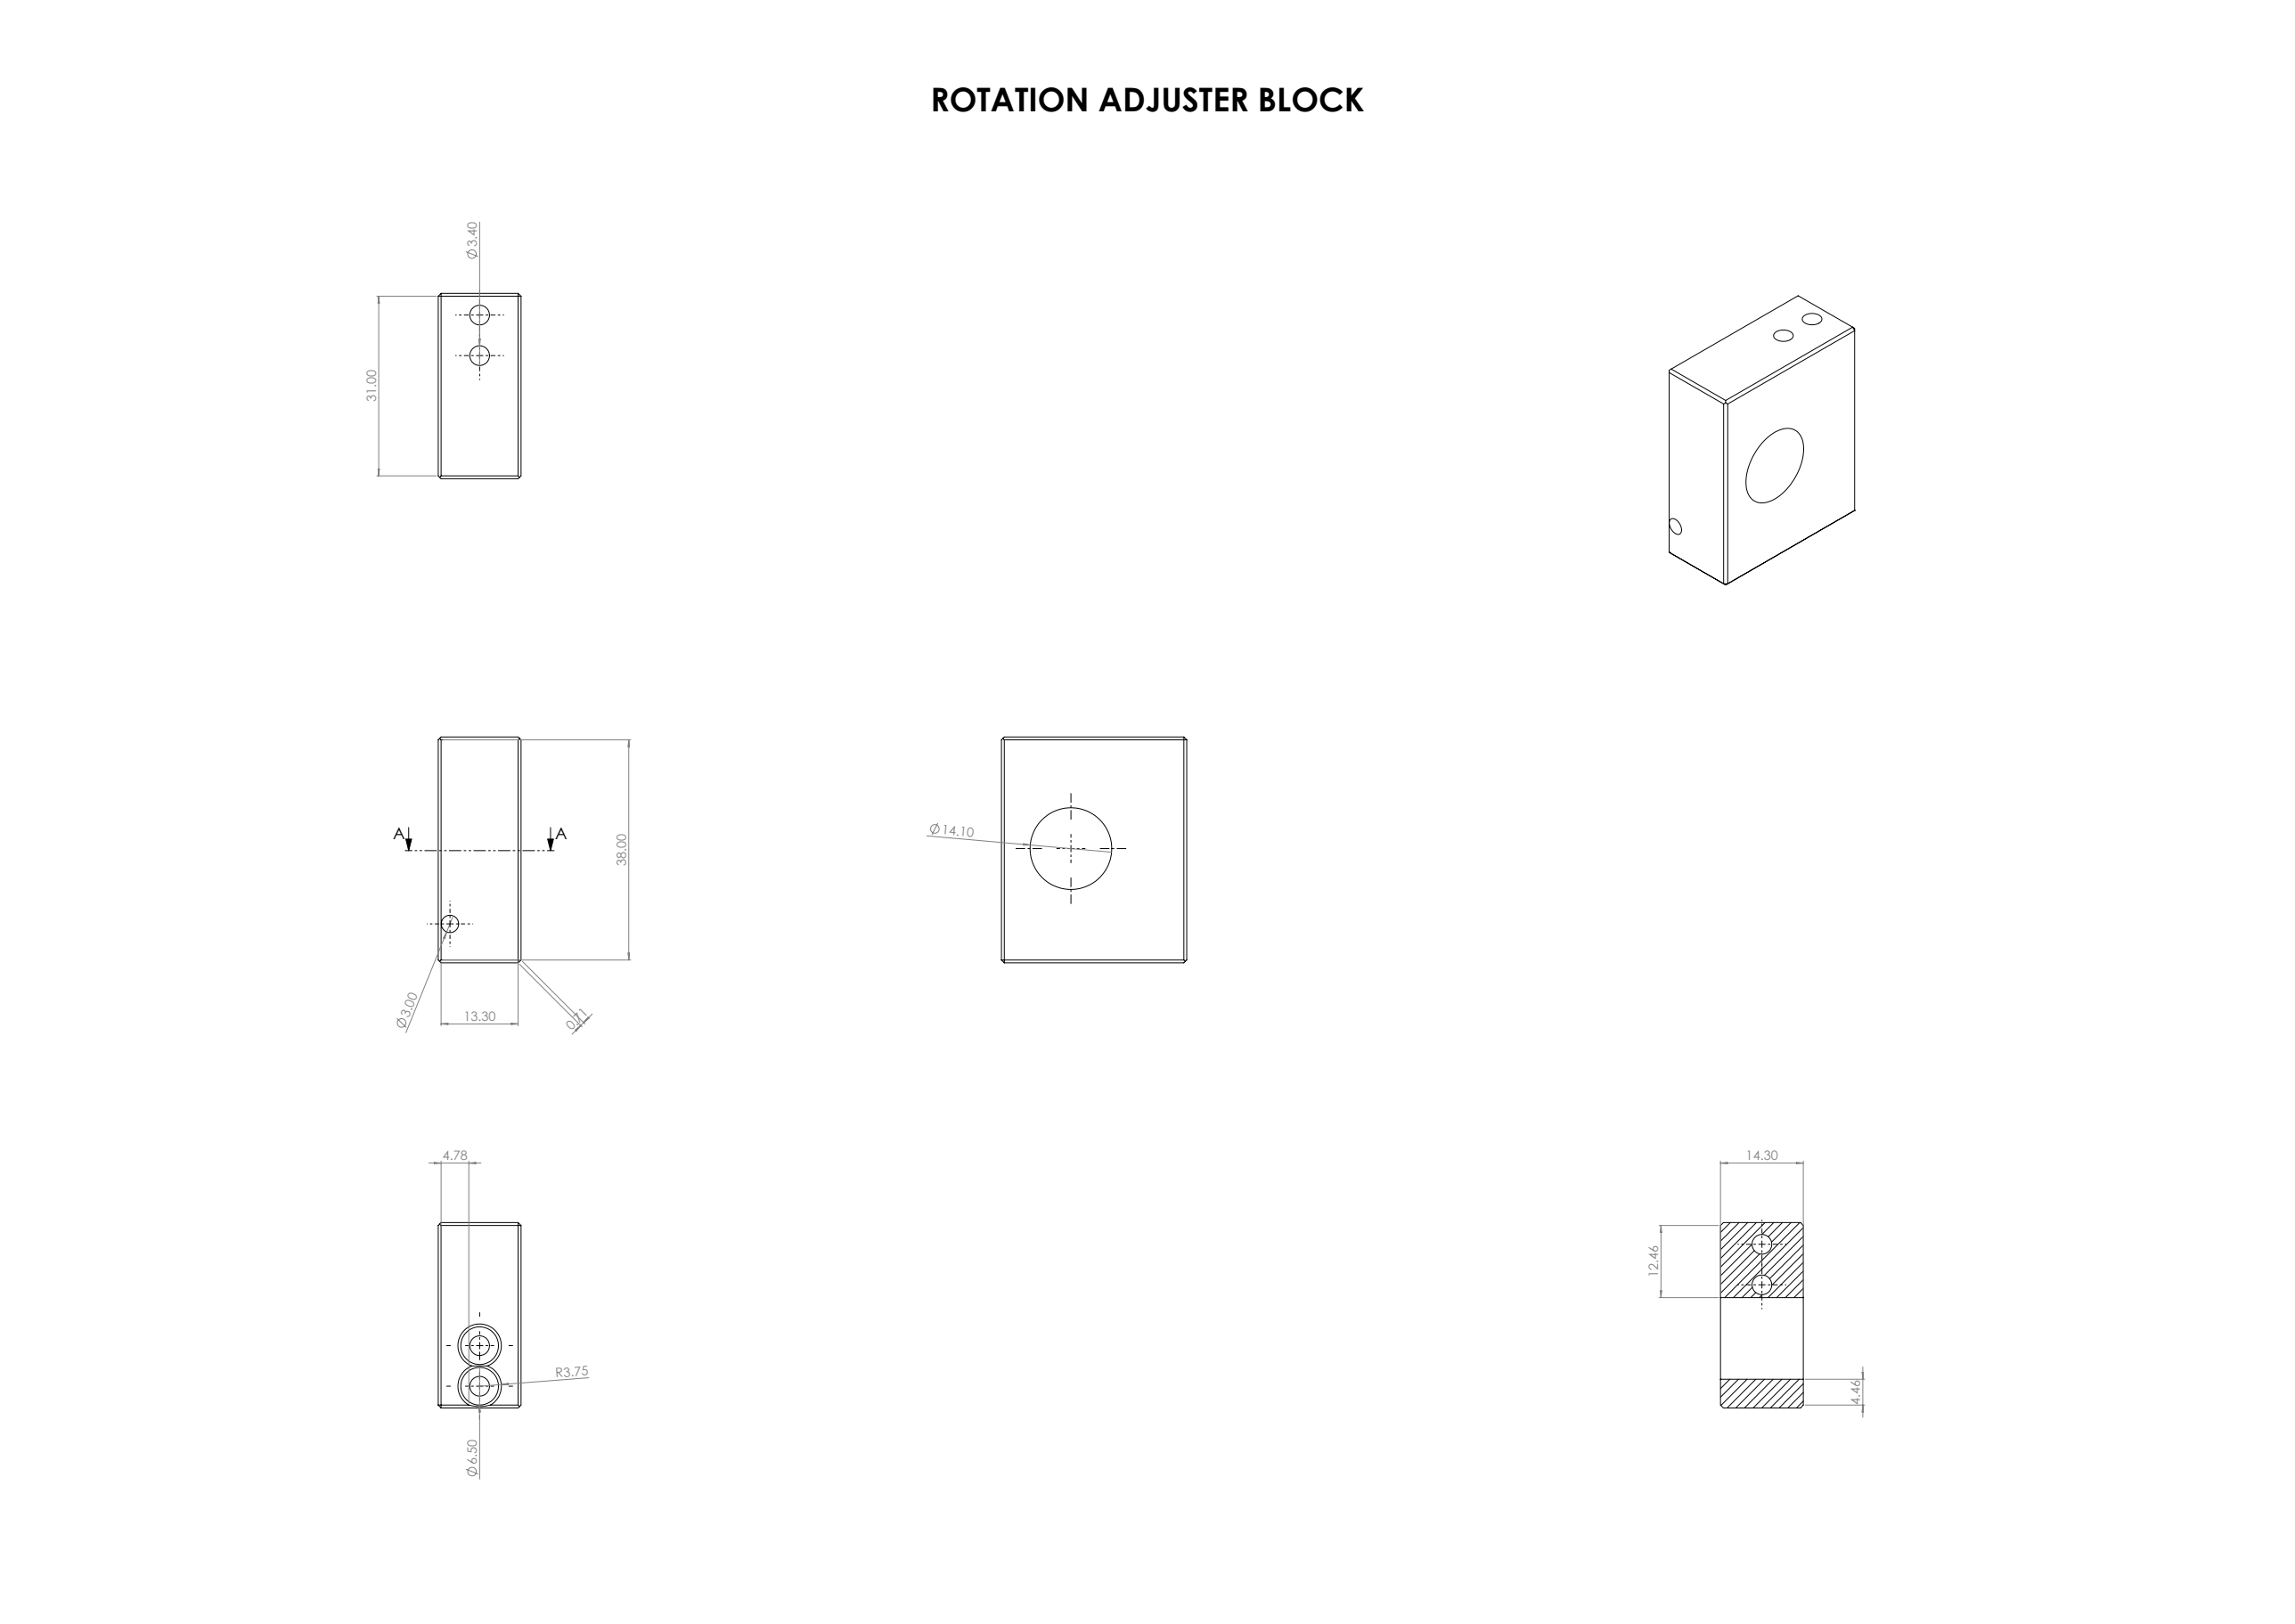
ISO-10303-21;
HEADER;
/* Generated by software containing ST-Developer
 * from STEP Tools, Inc. (www.steptools.com) 
 */

FILE_DESCRIPTION(
/* description */ (''),
/* implementation_level */ '2;1');

FILE_NAME(
/* name */ '04_Rotation_Adjuster_Block.step',
/* time_stamp */ '2026-10-21T01:56:51-07:00',
/* author */ (''),
/* organization */ (''),
/* preprocessor_version */ 'ST-DEVELOPER v20.2',
/* originating_system */ 'Autodesk Translation Framework v15.15.0.0',
/* authorisation */ '');

FILE_SCHEMA (('AUTOMOTIVE_DESIGN { 1 0 10303 214 3 1 1 }'));
ENDSEC;

DATA;
#10=MECHANICAL_DESIGN_GEOMETRIC_PRESENTATION_REPRESENTATION('',(#273),#82384);
#169=(
BOUNDED_CURVE()
B_SPLINE_CURVE(2,(#44591,#44592,#44593),.UNSPECIFIED.,.F.,.F.)
B_SPLINE_CURVE_WITH_KNOTS((3,3),(0.,0.380788655293197),.UNSPECIFIED.)
CURVE()
GEOMETRIC_REPRESENTATION_ITEM()
RATIONAL_B_SPLINE_CURVE((1.,1.,1.))
REPRESENTATION_ITEM('')
);
#235=SHAPE_REPRESENTATION_RELATIONSHIP('SRR','None',#82469,#254);
#254=ADVANCED_BREP_SHAPE_REPRESENTATION('',(#292),#82368);
#273=STYLED_ITEM('',(#82610),#292);
#292=MANIFOLD_SOLID_BREP('Body1',#30664);
#538=CYLINDRICAL_SURFACE('',#31720,3.25);
#539=CYLINDRICAL_SURFACE('',#31723,3.25);
#540=CYLINDRICAL_SURFACE('',#31755,1.7);
#541=CYLINDRICAL_SURFACE('',#31756,1.7);
#542=CYLINDRICAL_SURFACE('',#31757,1.5);
#543=CYLINDRICAL_SURFACE('',#31758,1.5);
#544=CYLINDRICAL_SURFACE('',#31761,4.5);
#545=CYLINDRICAL_SURFACE('',#31764,7.05);
#1402=CIRCLE('',#31712,3.75);
#1403=CIRCLE('',#31713,3.25);
#1404=CIRCLE('',#31714,3.75);
#1405=CIRCLE('',#31716,3.75);
#1406=CIRCLE('',#31717,3.25);
#1407=CIRCLE('',#31718,3.75);
#1408=CIRCLE('',#31719,3.75);
#1409=CIRCLE('',#31721,3.25);
#1410=CIRCLE('',#31724,3.25);
#1411=CIRCLE('',#31735,1.7);
#1412=CIRCLE('',#31736,1.7);
#1413=CIRCLE('',#31738,7.05);
#1414=CIRCLE('',#31739,4.5);
#1415=CIRCLE('',#31748,7.05);
#1416=CIRCLE('',#31750,1.5);
#1417=CIRCLE('',#31752,1.7);
#1418=CIRCLE('',#31754,1.7);
#1419=CIRCLE('',#31759,1.5);
#1420=CIRCLE('',#31762,4.5);
#2029=CONICAL_SURFACE('',#31711,3.5,0.785398163397442);
#2030=CONICAL_SURFACE('',#31715,3.5,0.785398163397442);
#2310=B_SPLINE_CURVE_WITH_KNOTS('',3,(#44570,#44571,#44572,#44573,#44574,
#44575),.UNSPECIFIED.,.F.,.F.,(4,2,4),(1.60159343096041,1.75059102484718,
1.89958861873394),.UNSPECIFIED.);
#2311=B_SPLINE_CURVE_WITH_KNOTS('',3,(#44727,#44728,#44729,#44730,#44731,
#44732,#44733,#44734,#44735,#44736),.UNSPECIFIED.,.F.,.F.,(4,2,2,2,4),(0.,
0.056990727183553,0.113981454367106,0.170945749207414,0.227910044047722),
 .UNSPECIFIED.);
#2312=B_SPLINE_CURVE_WITH_KNOTS('',3,(#44738,#44739,#44740,#44741,#44742,
#44743,#44744,#44745,#44746,#44747),.UNSPECIFIED.,.F.,.F.,(4,2,2,2,4),(0.683730132143166,
0.740694426983474,0.797658721823782,0.854649449007335,0.911640176190888),
 .UNSPECIFIED.);
#2313=B_SPLINE_CURVE_WITH_KNOTS('',3,(#44748,#44749,#44750,#44751,#44752,
#44753,#44754,#44755,#44756,#44757,#44758,#44759,#44760,#44761,#44762,#44763,
#44764,#44765),.UNSPECIFIED.,.F.,.F.,(4,2,2,2,2,2,2,2,4),(0.227910044047722,
0.28487433888803,0.341838633728338,0.398829360911891,0.455820088095444,
0.512810815278997,0.56980154246255,0.626765837302858,0.683730132143166),
 .UNSPECIFIED.);
#2314=B_SPLINE_CURVE_WITH_KNOTS('',3,(#44769,#44770,#44771,#44772,#44773,
#44774,#44775,#44776,#44777,#44778,#44779,#44780,#44781,#44782,#44783,#44784,
#44785,#44786,#44787,#44788,#44789,#44790,#44791,#44792,#44793,#44794),
 .UNSPECIFIED.,.F.,.F.,(4,2,2,2,2,2,2,2,2,2,2,2,4),(0.,0.056990727183553,
0.113981454367106,0.170945749207414,0.227910044047722,0.28487433888803,
0.341838633728338,0.398829360911891,0.455820088095444,0.512810815278997,
0.56980154246255,0.626765837302858,0.683730132143166),.UNSPECIFIED.);
#2315=B_SPLINE_CURVE_WITH_KNOTS('',3,(#44795,#44796,#44797,#44798,#44799,
#44800,#44801,#44802,#44803,#44804),.UNSPECIFIED.,.F.,.F.,(4,2,2,2,4),(0.683730132143166,
0.740694426983474,0.797658721823782,0.854649449007335,0.911640176190888),
 .UNSPECIFIED.);
#3434=FACE_BOUND('',#6058,.T.);
#3435=FACE_BOUND('',#6059,.T.);
#3436=FACE_BOUND('',#6061,.T.);
#3437=FACE_BOUND('',#6062,.T.);
#3438=FACE_BOUND('',#6071,.T.);
#3439=FACE_BOUND('',#6073,.T.);
#3440=FACE_BOUND('',#6075,.T.);
#3441=FACE_BOUND('',#6077,.T.);
#3442=FACE_BOUND('',#6084,.T.);
#4137=FACE_OUTER_BOUND('',#6043,.T.);
#4138=FACE_OUTER_BOUND('',#6044,.T.);
#4139=FACE_OUTER_BOUND('',#6045,.T.);
#4140=FACE_OUTER_BOUND('',#6046,.T.);
#4141=FACE_OUTER_BOUND('',#6047,.T.);
#4142=FACE_OUTER_BOUND('',#6048,.T.);
#4143=FACE_OUTER_BOUND('',#6049,.T.);
#4144=FACE_OUTER_BOUND('',#6050,.T.);
#4145=FACE_OUTER_BOUND('',#6051,.T.);
#4146=FACE_OUTER_BOUND('',#6052,.T.);
#4147=FACE_OUTER_BOUND('',#6053,.T.);
#4148=FACE_OUTER_BOUND('',#6054,.T.);
#4149=FACE_OUTER_BOUND('',#6055,.T.);
#4150=FACE_OUTER_BOUND('',#6056,.T.);
#4151=FACE_OUTER_BOUND('',#6057,.T.);
#4152=FACE_OUTER_BOUND('',#6060,.T.);
#4153=FACE_OUTER_BOUND('',#6063,.T.);
#4154=FACE_OUTER_BOUND('',#6064,.T.);
#4155=FACE_OUTER_BOUND('',#6065,.T.);
#4156=FACE_OUTER_BOUND('',#6066,.T.);
#4157=FACE_OUTER_BOUND('',#6067,.T.);
#4158=FACE_OUTER_BOUND('',#6068,.T.);
#4159=FACE_OUTER_BOUND('',#6069,.T.);
#4160=FACE_OUTER_BOUND('',#6070,.T.);
#4161=FACE_OUTER_BOUND('',#6072,.T.);
#4162=FACE_OUTER_BOUND('',#6074,.T.);
#4163=FACE_OUTER_BOUND('',#6076,.T.);
#4164=FACE_OUTER_BOUND('',#6078,.T.);
#4165=FACE_OUTER_BOUND('',#6079,.T.);
#4166=FACE_OUTER_BOUND('',#6080,.T.);
#4167=FACE_OUTER_BOUND('',#6081,.T.);
#4168=FACE_OUTER_BOUND('',#6082,.T.);
#4169=FACE_OUTER_BOUND('',#6083,.T.);
#4170=FACE_OUTER_BOUND('',#6085,.T.);
#4171=FACE_OUTER_BOUND('',#6086,.T.);
#4172=FACE_OUTER_BOUND('',#6087,.T.);
#6043=EDGE_LOOP('',(#21929,#21930,#21931,#21932,#21933,#21934));
#6044=EDGE_LOOP('',(#21935,#21936,#21937,#21938,#21939,#21940,#21941,#21942));
#6045=EDGE_LOOP('',(#21943,#21944,#21945,#21946));
#6046=EDGE_LOOP('',(#21947,#21948,#21949,#21950,#21951,#21952,#21953));
#6047=EDGE_LOOP('',(#21954,#21955,#21956,#21957));
#6048=EDGE_LOOP('',(#21958,#21959,#21960));
#6049=EDGE_LOOP('',(#21961,#21962,#21963));
#6050=EDGE_LOOP('',(#21964,#21965,#21966,#21967));
#6051=EDGE_LOOP('',(#21968,#21969,#21970,#21971,#21972));
#6052=EDGE_LOOP('',(#21973,#21974,#21975));
#6053=EDGE_LOOP('',(#21976,#21977,#21978,#21979,#21980));
#6054=EDGE_LOOP('',(#21981,#21982,#21983,#21984));
#6055=EDGE_LOOP('',(#21985,#21986,#21987,#21988,#21989));
#6056=EDGE_LOOP('',(#21990,#21991,#21992,#21993,#21994));
#6057=EDGE_LOOP('',(#21995,#21996,#21997,#21998));
#6058=EDGE_LOOP('',(#21999));
#6059=EDGE_LOOP('',(#22000));
#6060=EDGE_LOOP('',(#22001,#22002,#22003,#22004));
#6061=EDGE_LOOP('',(#22005));
#6062=EDGE_LOOP('',(#22006));
#6063=EDGE_LOOP('',(#22007,#22008,#22009,#22010,#22011,#22012));
#6064=EDGE_LOOP('',(#22013,#22014,#22015,#22016,#22017));
#6065=EDGE_LOOP('',(#22018,#22019,#22020,#22021));
#6066=EDGE_LOOP('',(#22022,#22023,#22024));
#6067=EDGE_LOOP('',(#22025,#22026,#22027,#22028,#22029));
#6068=EDGE_LOOP('',(#22030,#22031,#22032,#22033,#22034,#22035));
#6069=EDGE_LOOP('',(#22036,#22037,#22038,#22039,#22040));
#6070=EDGE_LOOP('',(#22041,#22042,#22043,#22044));
#6071=EDGE_LOOP('',(#22045));
#6072=EDGE_LOOP('',(#22046,#22047,#22048,#22049));
#6073=EDGE_LOOP('',(#22050));
#6074=EDGE_LOOP('',(#22051));
#6075=EDGE_LOOP('',(#22052));
#6076=EDGE_LOOP('',(#22053));
#6077=EDGE_LOOP('',(#22054));
#6078=EDGE_LOOP('',(#22055,#22056,#22057,#22058));
#6079=EDGE_LOOP('',(#22059,#22060,#22061,#22062));
#6080=EDGE_LOOP('',(#22063,#22064,#22065,#22066,#22067,#22068));
#6081=EDGE_LOOP('',(#22069,#22070,#22071,#22072,#22073));
#6082=EDGE_LOOP('',(#22074));
#6083=EDGE_LOOP('',(#22075,#22076,#22077,#22078,#22079,#22080,#22081,#22082,
#22083));
#6084=EDGE_LOOP('',(#22084,#22085));
#6085=EDGE_LOOP('',(#22086));
#6086=EDGE_LOOP('',(#22087,#22088,#22089,#22090));
#6087=EDGE_LOOP('',(#22091,#22092,#22093,#22094,#22095,#22096,#22097,#22098,
#22099,#22100));
#8112=LINE('',#44579,#10418);
#8113=LINE('',#44586,#10419);
#8114=LINE('',#44597,#10420);
#8115=LINE('',#44601,#10421);
#8116=LINE('',#44603,#10422);
#8117=LINE('',#44605,#10423);
#8118=LINE('',#44607,#10424);
#8119=LINE('',#44609,#10425);
#8120=LINE('',#44610,#10426);
#8121=LINE('',#44613,#10427);
#8122=LINE('',#44617,#10428);
#8123=LINE('',#44618,#10429);
#8124=LINE('',#44622,#10430);
#8125=LINE('',#44624,#10431);
#8126=LINE('',#44625,#10432);
#8127=LINE('',#44627,#10433);
#8128=LINE('',#44628,#10434);
#8129=LINE('',#44632,#10435);
#8130=LINE('',#44633,#10436);
#8131=LINE('',#44635,#10437);
#8132=LINE('',#44636,#10438);
#8133=LINE('',#44640,#10439);
#8134=LINE('',#44642,#10440);
#8135=LINE('',#44643,#10441);
#8136=LINE('',#44645,#10442);
#8137=LINE('',#44647,#10443);
#8138=LINE('',#44648,#10444);
#8139=LINE('',#44650,#10445);
#8140=LINE('',#44651,#10446);
#8141=LINE('',#44655,#10447);
#8142=LINE('',#44656,#10448);
#8143=LINE('',#44658,#10449);
#8144=LINE('',#44659,#10450);
#8145=LINE('',#44663,#10451);
#8146=LINE('',#44664,#10452);
#8147=LINE('',#44666,#10453);
#8148=LINE('',#44667,#10454);
#8149=LINE('',#44669,#10455);
#8150=LINE('',#44675,#10456);
#8151=LINE('',#44682,#10457);
#8152=LINE('',#44684,#10458);
#8153=LINE('',#44685,#10459);
#8154=LINE('',#44688,#10460);
#8155=LINE('',#44690,#10461);
#8156=LINE('',#44691,#10462);
#8157=LINE('',#44695,#10463);
#8158=LINE('',#44696,#10464);
#8159=LINE('',#44698,#10465);
#8160=LINE('',#44699,#10466);
#8161=LINE('',#44702,#10467);
#8162=LINE('',#44703,#10468);
#8163=LINE('',#44705,#10469);
#8164=LINE('',#44706,#10470);
#8165=LINE('',#44720,#10471);
#8166=LINE('',#44722,#10472);
#8167=LINE('',#44725,#10473);
#8168=LINE('',#44806,#10474);
#8169=LINE('',#44810,#10475);
#8170=LINE('',#44812,#10476);
#8171=LINE('',#44816,#10477);
#10418=VECTOR('',#35789,3.5);
#10419=VECTOR('',#35798,3.5);
#10420=VECTOR('',#35807,3.25);
#10421=VECTOR('',#35812,10.);
#10422=VECTOR('',#35813,10.);
#10423=VECTOR('',#35814,10.);
#10424=VECTOR('',#35815,10.);
#10425=VECTOR('',#35816,10.);
#10426=VECTOR('',#35817,10.);
#10427=VECTOR('',#35820,3.25);
#10428=VECTOR('',#35825,10.);
#10429=VECTOR('',#35826,10.);
#10430=VECTOR('',#35829,10.);
#10431=VECTOR('',#35830,10.);
#10432=VECTOR('',#35831,10.);
#10433=VECTOR('',#35834,10.);
#10434=VECTOR('',#35835,10.);
#10435=VECTOR('',#35838,10.);
#10436=VECTOR('',#35839,10.);
#10437=VECTOR('',#35840,10.);
#10438=VECTOR('',#35841,10.);
#10439=VECTOR('',#35844,10.);
#10440=VECTOR('',#35845,10.);
#10441=VECTOR('',#35846,10.);
#10442=VECTOR('',#35849,10.);
#10443=VECTOR('',#35850,10.);
#10444=VECTOR('',#35851,10.);
#10445=VECTOR('',#35854,10.);
#10446=VECTOR('',#35855,10.);
#10447=VECTOR('',#35858,10.);
#10448=VECTOR('',#35859,10.);
#10449=VECTOR('',#35860,10.);
#10450=VECTOR('',#35861,10.);
#10451=VECTOR('',#35864,10.);
#10452=VECTOR('',#35865,10.);
#10453=VECTOR('',#35866,10.);
#10454=VECTOR('',#35867,10.);
#10455=VECTOR('',#35870,10.);
#10456=VECTOR('',#35877,10.);
#10457=VECTOR('',#35884,10.);
#10458=VECTOR('',#35885,10.);
#10459=VECTOR('',#35886,10.);
#10460=VECTOR('',#35889,10.);
#10461=VECTOR('',#35890,10.);
#10462=VECTOR('',#35891,10.);
#10463=VECTOR('',#35896,10.);
#10464=VECTOR('',#35897,10.);
#10465=VECTOR('',#35900,10.);
#10466=VECTOR('',#35901,10.);
#10467=VECTOR('',#35904,10.);
#10468=VECTOR('',#35905,10.);
#10469=VECTOR('',#35908,10.);
#10470=VECTOR('',#35909,10.);
#10471=VECTOR('',#35928,1.7);
#10472=VECTOR('',#35931,1.7);
#10473=VECTOR('',#35934,1.5);
#10474=VECTOR('',#35937,1.5);
#10475=VECTOR('',#35944,4.5);
#10476=VECTOR('',#35945,4.5);
#10477=VECTOR('',#35952,7.05);
#12816=VERTEX_POINT('',#44568);
#12817=VERTEX_POINT('',#44569);
#12818=VERTEX_POINT('',#44576);
#12819=VERTEX_POINT('',#44578);
#12820=VERTEX_POINT('',#44583);
#12821=VERTEX_POINT('',#44585);
#12822=VERTEX_POINT('',#44588);
#12823=VERTEX_POINT('',#44590);
#12824=VERTEX_POINT('',#44596);
#12825=VERTEX_POINT('',#44600);
#12826=VERTEX_POINT('',#44602);
#12827=VERTEX_POINT('',#44604);
#12828=VERTEX_POINT('',#44606);
#12829=VERTEX_POINT('',#44608);
#12830=VERTEX_POINT('',#44612);
#12831=VERTEX_POINT('',#44616);
#12832=VERTEX_POINT('',#44620);
#12833=VERTEX_POINT('',#44621);
#12834=VERTEX_POINT('',#44623);
#12835=VERTEX_POINT('',#44630);
#12836=VERTEX_POINT('',#44631);
#12837=VERTEX_POINT('',#44634);
#12838=VERTEX_POINT('',#44638);
#12839=VERTEX_POINT('',#44639);
#12840=VERTEX_POINT('',#44641);
#12841=VERTEX_POINT('',#44646);
#12842=VERTEX_POINT('',#44653);
#12843=VERTEX_POINT('',#44654);
#12844=VERTEX_POINT('',#44657);
#12845=VERTEX_POINT('',#44661);
#12846=VERTEX_POINT('',#44662);
#12847=VERTEX_POINT('',#44665);
#12848=VERTEX_POINT('',#44670);
#12849=VERTEX_POINT('',#44672);
#12850=VERTEX_POINT('',#44676);
#12851=VERTEX_POINT('',#44678);
#12852=VERTEX_POINT('',#44681);
#12853=VERTEX_POINT('',#44683);
#12854=VERTEX_POINT('',#44687);
#12855=VERTEX_POINT('',#44689);
#12856=VERTEX_POINT('',#44694);
#12857=VERTEX_POINT('',#44701);
#12858=VERTEX_POINT('',#44708);
#12859=VERTEX_POINT('',#44711);
#12860=VERTEX_POINT('',#44714);
#12861=VERTEX_POINT('',#44717);
#12862=VERTEX_POINT('',#44724);
#12863=VERTEX_POINT('',#44726);
#12864=VERTEX_POINT('',#44737);
#12865=VERTEX_POINT('',#44767);
#12866=VERTEX_POINT('',#44768);
#12867=VERTEX_POINT('',#44805);
#12868=VERTEX_POINT('',#44811);
#16186=EDGE_CURVE('',#12816,#12817,#2310,.T.);
#16187=EDGE_CURVE('',#12817,#12818,#1402,.T.);
#16188=EDGE_CURVE('',#12818,#12819,#8112,.T.);
#16189=EDGE_CURVE('',#12819,#12819,#1403,.T.);
#16190=EDGE_CURVE('',#12818,#12816,#1404,.T.);
#16191=EDGE_CURVE('',#12816,#12820,#1405,.T.);
#16192=EDGE_CURVE('',#12820,#12821,#8113,.T.);
#16193=EDGE_CURVE('',#12821,#12821,#1406,.T.);
#16194=EDGE_CURVE('',#12820,#12822,#1407,.T.);
#16195=EDGE_CURVE('',#12822,#12823,#169,.T.);
#16196=EDGE_CURVE('',#12823,#12817,#1408,.T.);
#16197=EDGE_CURVE('',#12819,#12824,#8114,.T.);
#16198=EDGE_CURVE('',#12824,#12824,#1409,.T.);
#16199=EDGE_CURVE('',#12822,#12825,#8115,.T.);
#16200=EDGE_CURVE('',#12825,#12826,#8116,.T.);
#16201=EDGE_CURVE('',#12826,#12827,#8117,.T.);
#16202=EDGE_CURVE('',#12828,#12827,#8118,.T.);
#16203=EDGE_CURVE('',#12828,#12829,#8119,.T.);
#16204=EDGE_CURVE('',#12829,#12823,#8120,.T.);
#16205=EDGE_CURVE('',#12821,#12830,#8121,.T.);
#16206=EDGE_CURVE('',#12830,#12830,#1410,.T.);
#16207=EDGE_CURVE('',#12831,#12825,#8122,.T.);
#16208=EDGE_CURVE('',#12826,#12831,#8123,.T.);
#16209=EDGE_CURVE('',#12832,#12833,#8124,.T.);
#16210=EDGE_CURVE('',#12834,#12832,#8125,.T.);
#16211=EDGE_CURVE('',#12833,#12834,#8126,.T.);
#16212=EDGE_CURVE('',#12831,#12834,#8127,.T.);
#16213=EDGE_CURVE('',#12832,#12826,#8128,.T.);
#16214=EDGE_CURVE('',#12835,#12836,#8129,.T.);
#16215=EDGE_CURVE('',#12836,#12833,#8130,.T.);
#16216=EDGE_CURVE('',#12834,#12837,#8131,.T.);
#16217=EDGE_CURVE('',#12837,#12835,#8132,.T.);
#16218=EDGE_CURVE('',#12838,#12839,#8133,.T.);
#16219=EDGE_CURVE('',#12840,#12838,#8134,.T.);
#16220=EDGE_CURVE('',#12839,#12840,#8135,.T.);
#16221=EDGE_CURVE('',#12827,#12840,#8136,.T.);
#16222=EDGE_CURVE('',#12838,#12841,#8137,.T.);
#16223=EDGE_CURVE('',#12841,#12828,#8138,.T.);
#16224=EDGE_CURVE('',#12833,#12839,#8139,.T.);
#16225=EDGE_CURVE('',#12840,#12832,#8140,.T.);
#16226=EDGE_CURVE('',#12842,#12843,#8141,.T.);
#16227=EDGE_CURVE('',#12843,#12838,#8142,.T.);
#16228=EDGE_CURVE('',#12839,#12844,#8143,.T.);
#16229=EDGE_CURVE('',#12844,#12842,#8144,.T.);
#16230=EDGE_CURVE('',#12845,#12846,#8145,.T.);
#16231=EDGE_CURVE('',#12846,#12831,#8146,.T.);
#16232=EDGE_CURVE('',#12825,#12847,#8147,.T.);
#16233=EDGE_CURVE('',#12847,#12845,#8148,.T.);
#16234=EDGE_CURVE('',#12844,#12836,#8149,.T.);
#16235=EDGE_CURVE('',#12848,#12848,#1411,.T.);
#16236=EDGE_CURVE('',#12849,#12849,#1412,.T.);
#16237=EDGE_CURVE('',#12837,#12846,#8150,.T.);
#16238=EDGE_CURVE('',#12850,#12850,#1413,.T.);
#16239=EDGE_CURVE('',#12851,#12851,#1414,.T.);
#16240=EDGE_CURVE('',#12852,#12845,#8151,.T.);
#16241=EDGE_CURVE('',#12852,#12853,#8152,.T.);
#16242=EDGE_CURVE('',#12853,#12835,#8153,.T.);
#16243=EDGE_CURVE('',#12847,#12854,#8154,.T.);
#16244=EDGE_CURVE('',#12854,#12855,#8155,.T.);
#16245=EDGE_CURVE('',#12855,#12852,#8156,.T.);
#16246=EDGE_CURVE('',#12856,#12854,#8157,.T.);
#16247=EDGE_CURVE('',#12855,#12856,#8158,.T.);
#16248=EDGE_CURVE('',#12841,#12856,#8159,.T.);
#16249=EDGE_CURVE('',#12854,#12829,#8160,.T.);
#16250=EDGE_CURVE('',#12853,#12857,#8161,.T.);
#16251=EDGE_CURVE('',#12857,#12842,#8162,.T.);
#16252=EDGE_CURVE('',#12857,#12855,#8163,.T.);
#16253=EDGE_CURVE('',#12856,#12843,#8164,.T.);
#16254=EDGE_CURVE('',#12858,#12858,#1415,.T.);
#16255=EDGE_CURVE('',#12859,#12859,#1416,.T.);
#16256=EDGE_CURVE('',#12860,#12860,#1417,.T.);
#16257=EDGE_CURVE('',#12861,#12861,#1418,.T.);
#16258=EDGE_CURVE('',#12860,#12849,#8165,.T.);
#16259=EDGE_CURVE('',#12861,#12848,#8166,.T.);
#16260=EDGE_CURVE('',#12859,#12862,#8167,.T.);
#16261=EDGE_CURVE('',#12863,#12862,#2311,.T.);
#16262=EDGE_CURVE('',#12864,#12863,#2312,.T.);
#16263=EDGE_CURVE('',#12862,#12864,#2313,.T.);
#16264=EDGE_CURVE('',#12865,#12866,#2314,.T.);
#16265=EDGE_CURVE('',#12866,#12865,#2315,.T.);
#16266=EDGE_CURVE('',#12866,#12867,#8168,.T.);
#16267=EDGE_CURVE('',#12867,#12867,#1419,.T.);
#16268=EDGE_CURVE('',#12851,#12862,#8169,.T.);
#16269=EDGE_CURVE('',#12864,#12868,#8170,.T.);
#16270=EDGE_CURVE('',#12868,#12868,#1420,.T.);
#16271=EDGE_CURVE('',#12858,#12850,#8171,.T.);
#21929=ORIENTED_EDGE('',*,*,#16186,.T.);
#21930=ORIENTED_EDGE('',*,*,#16187,.T.);
#21931=ORIENTED_EDGE('',*,*,#16188,.T.);
#21932=ORIENTED_EDGE('',*,*,#16189,.T.);
#21933=ORIENTED_EDGE('',*,*,#16188,.F.);
#21934=ORIENTED_EDGE('',*,*,#16190,.T.);
#21935=ORIENTED_EDGE('',*,*,#16186,.F.);
#21936=ORIENTED_EDGE('',*,*,#16191,.T.);
#21937=ORIENTED_EDGE('',*,*,#16192,.T.);
#21938=ORIENTED_EDGE('',*,*,#16193,.T.);
#21939=ORIENTED_EDGE('',*,*,#16192,.F.);
#21940=ORIENTED_EDGE('',*,*,#16194,.T.);
#21941=ORIENTED_EDGE('',*,*,#16195,.T.);
#21942=ORIENTED_EDGE('',*,*,#16196,.T.);
#21943=ORIENTED_EDGE('',*,*,#16189,.F.);
#21944=ORIENTED_EDGE('',*,*,#16197,.T.);
#21945=ORIENTED_EDGE('',*,*,#16198,.T.);
#21946=ORIENTED_EDGE('',*,*,#16197,.F.);
#21947=ORIENTED_EDGE('',*,*,#16195,.F.);
#21948=ORIENTED_EDGE('',*,*,#16199,.T.);
#21949=ORIENTED_EDGE('',*,*,#16200,.T.);
#21950=ORIENTED_EDGE('',*,*,#16201,.T.);
#21951=ORIENTED_EDGE('',*,*,#16202,.F.);
#21952=ORIENTED_EDGE('',*,*,#16203,.T.);
#21953=ORIENTED_EDGE('',*,*,#16204,.T.);
#21954=ORIENTED_EDGE('',*,*,#16193,.F.);
#21955=ORIENTED_EDGE('',*,*,#16205,.T.);
#21956=ORIENTED_EDGE('',*,*,#16206,.T.);
#21957=ORIENTED_EDGE('',*,*,#16205,.F.);
#21958=ORIENTED_EDGE('',*,*,#16207,.F.);
#21959=ORIENTED_EDGE('',*,*,#16208,.F.);
#21960=ORIENTED_EDGE('',*,*,#16200,.F.);
#21961=ORIENTED_EDGE('',*,*,#16209,.F.);
#21962=ORIENTED_EDGE('',*,*,#16210,.F.);
#21963=ORIENTED_EDGE('',*,*,#16211,.F.);
#21964=ORIENTED_EDGE('',*,*,#16208,.T.);
#21965=ORIENTED_EDGE('',*,*,#16212,.T.);
#21966=ORIENTED_EDGE('',*,*,#16210,.T.);
#21967=ORIENTED_EDGE('',*,*,#16213,.T.);
#21968=ORIENTED_EDGE('',*,*,#16214,.T.);
#21969=ORIENTED_EDGE('',*,*,#16215,.T.);
#21970=ORIENTED_EDGE('',*,*,#16211,.T.);
#21971=ORIENTED_EDGE('',*,*,#16216,.T.);
#21972=ORIENTED_EDGE('',*,*,#16217,.T.);
#21973=ORIENTED_EDGE('',*,*,#16218,.F.);
#21974=ORIENTED_EDGE('',*,*,#16219,.F.);
#21975=ORIENTED_EDGE('',*,*,#16220,.F.);
#21976=ORIENTED_EDGE('',*,*,#16202,.T.);
#21977=ORIENTED_EDGE('',*,*,#16221,.T.);
#21978=ORIENTED_EDGE('',*,*,#16219,.T.);
#21979=ORIENTED_EDGE('',*,*,#16222,.T.);
#21980=ORIENTED_EDGE('',*,*,#16223,.T.);
#21981=ORIENTED_EDGE('',*,*,#16209,.T.);
#21982=ORIENTED_EDGE('',*,*,#16224,.T.);
#21983=ORIENTED_EDGE('',*,*,#16220,.T.);
#21984=ORIENTED_EDGE('',*,*,#16225,.T.);
#21985=ORIENTED_EDGE('',*,*,#16226,.T.);
#21986=ORIENTED_EDGE('',*,*,#16227,.T.);
#21987=ORIENTED_EDGE('',*,*,#16218,.T.);
#21988=ORIENTED_EDGE('',*,*,#16228,.T.);
#21989=ORIENTED_EDGE('',*,*,#16229,.T.);
#21990=ORIENTED_EDGE('',*,*,#16230,.T.);
#21991=ORIENTED_EDGE('',*,*,#16231,.T.);
#21992=ORIENTED_EDGE('',*,*,#16207,.T.);
#21993=ORIENTED_EDGE('',*,*,#16232,.T.);
#21994=ORIENTED_EDGE('',*,*,#16233,.T.);
#21995=ORIENTED_EDGE('',*,*,#16228,.F.);
#21996=ORIENTED_EDGE('',*,*,#16224,.F.);
#21997=ORIENTED_EDGE('',*,*,#16215,.F.);
#21998=ORIENTED_EDGE('',*,*,#16234,.F.);
#21999=ORIENTED_EDGE('',*,*,#16235,.T.);
#22000=ORIENTED_EDGE('',*,*,#16236,.T.);
#22001=ORIENTED_EDGE('',*,*,#16216,.F.);
#22002=ORIENTED_EDGE('',*,*,#16212,.F.);
#22003=ORIENTED_EDGE('',*,*,#16231,.F.);
#22004=ORIENTED_EDGE('',*,*,#16237,.F.);
#22005=ORIENTED_EDGE('',*,*,#16238,.T.);
#22006=ORIENTED_EDGE('',*,*,#16239,.T.);
#22007=ORIENTED_EDGE('',*,*,#16217,.F.);
#22008=ORIENTED_EDGE('',*,*,#16237,.T.);
#22009=ORIENTED_EDGE('',*,*,#16230,.F.);
#22010=ORIENTED_EDGE('',*,*,#16240,.F.);
#22011=ORIENTED_EDGE('',*,*,#16241,.T.);
#22012=ORIENTED_EDGE('',*,*,#16242,.T.);
#22013=ORIENTED_EDGE('',*,*,#16233,.F.);
#22014=ORIENTED_EDGE('',*,*,#16243,.T.);
#22015=ORIENTED_EDGE('',*,*,#16244,.T.);
#22016=ORIENTED_EDGE('',*,*,#16245,.T.);
#22017=ORIENTED_EDGE('',*,*,#16240,.T.);
#22018=ORIENTED_EDGE('',*,*,#16201,.F.);
#22019=ORIENTED_EDGE('',*,*,#16213,.F.);
#22020=ORIENTED_EDGE('',*,*,#16225,.F.);
#22021=ORIENTED_EDGE('',*,*,#16221,.F.);
#22022=ORIENTED_EDGE('',*,*,#16244,.F.);
#22023=ORIENTED_EDGE('',*,*,#16246,.F.);
#22024=ORIENTED_EDGE('',*,*,#16247,.F.);
#22025=ORIENTED_EDGE('',*,*,#16223,.F.);
#22026=ORIENTED_EDGE('',*,*,#16248,.T.);
#22027=ORIENTED_EDGE('',*,*,#16246,.T.);
#22028=ORIENTED_EDGE('',*,*,#16249,.T.);
#22029=ORIENTED_EDGE('',*,*,#16203,.F.);
#22030=ORIENTED_EDGE('',*,*,#16229,.F.);
#22031=ORIENTED_EDGE('',*,*,#16234,.T.);
#22032=ORIENTED_EDGE('',*,*,#16214,.F.);
#22033=ORIENTED_EDGE('',*,*,#16242,.F.);
#22034=ORIENTED_EDGE('',*,*,#16250,.T.);
#22035=ORIENTED_EDGE('',*,*,#16251,.T.);
#22036=ORIENTED_EDGE('',*,*,#16226,.F.);
#22037=ORIENTED_EDGE('',*,*,#16251,.F.);
#22038=ORIENTED_EDGE('',*,*,#16252,.T.);
#22039=ORIENTED_EDGE('',*,*,#16247,.T.);
#22040=ORIENTED_EDGE('',*,*,#16253,.T.);
#22041=ORIENTED_EDGE('',*,*,#16227,.F.);
#22042=ORIENTED_EDGE('',*,*,#16253,.F.);
#22043=ORIENTED_EDGE('',*,*,#16248,.F.);
#22044=ORIENTED_EDGE('',*,*,#16222,.F.);
#22045=ORIENTED_EDGE('',*,*,#16254,.T.);
#22046=ORIENTED_EDGE('',*,*,#16245,.F.);
#22047=ORIENTED_EDGE('',*,*,#16252,.F.);
#22048=ORIENTED_EDGE('',*,*,#16250,.F.);
#22049=ORIENTED_EDGE('',*,*,#16241,.F.);
#22050=ORIENTED_EDGE('',*,*,#16255,.T.);
#22051=ORIENTED_EDGE('',*,*,#16206,.F.);
#22052=ORIENTED_EDGE('',*,*,#16256,.F.);
#22053=ORIENTED_EDGE('',*,*,#16198,.F.);
#22054=ORIENTED_EDGE('',*,*,#16257,.F.);
#22055=ORIENTED_EDGE('',*,*,#16256,.T.);
#22056=ORIENTED_EDGE('',*,*,#16258,.T.);
#22057=ORIENTED_EDGE('',*,*,#16236,.F.);
#22058=ORIENTED_EDGE('',*,*,#16258,.F.);
#22059=ORIENTED_EDGE('',*,*,#16257,.T.);
#22060=ORIENTED_EDGE('',*,*,#16259,.T.);
#22061=ORIENTED_EDGE('',*,*,#16235,.F.);
#22062=ORIENTED_EDGE('',*,*,#16259,.F.);
#22063=ORIENTED_EDGE('',*,*,#16255,.F.);
#22064=ORIENTED_EDGE('',*,*,#16260,.T.);
#22065=ORIENTED_EDGE('',*,*,#16261,.F.);
#22066=ORIENTED_EDGE('',*,*,#16262,.F.);
#22067=ORIENTED_EDGE('',*,*,#16263,.F.);
#22068=ORIENTED_EDGE('',*,*,#16260,.F.);
#22069=ORIENTED_EDGE('',*,*,#16264,.F.);
#22070=ORIENTED_EDGE('',*,*,#16265,.F.);
#22071=ORIENTED_EDGE('',*,*,#16266,.T.);
#22072=ORIENTED_EDGE('',*,*,#16267,.T.);
#22073=ORIENTED_EDGE('',*,*,#16266,.F.);
#22074=ORIENTED_EDGE('',*,*,#16267,.F.);
#22075=ORIENTED_EDGE('',*,*,#16239,.F.);
#22076=ORIENTED_EDGE('',*,*,#16268,.T.);
#22077=ORIENTED_EDGE('',*,*,#16263,.T.);
#22078=ORIENTED_EDGE('',*,*,#16269,.T.);
#22079=ORIENTED_EDGE('',*,*,#16270,.T.);
#22080=ORIENTED_EDGE('',*,*,#16269,.F.);
#22081=ORIENTED_EDGE('',*,*,#16262,.T.);
#22082=ORIENTED_EDGE('',*,*,#16261,.T.);
#22083=ORIENTED_EDGE('',*,*,#16268,.F.);
#22084=ORIENTED_EDGE('',*,*,#16264,.T.);
#22085=ORIENTED_EDGE('',*,*,#16265,.T.);
#22086=ORIENTED_EDGE('',*,*,#16270,.F.);
#22087=ORIENTED_EDGE('',*,*,#16254,.F.);
#22088=ORIENTED_EDGE('',*,*,#16271,.T.);
#22089=ORIENTED_EDGE('',*,*,#16238,.F.);
#22090=ORIENTED_EDGE('',*,*,#16271,.F.);
#22091=ORIENTED_EDGE('',*,*,#16187,.F.);
#22092=ORIENTED_EDGE('',*,*,#16196,.F.);
#22093=ORIENTED_EDGE('',*,*,#16204,.F.);
#22094=ORIENTED_EDGE('',*,*,#16249,.F.);
#22095=ORIENTED_EDGE('',*,*,#16243,.F.);
#22096=ORIENTED_EDGE('',*,*,#16232,.F.);
#22097=ORIENTED_EDGE('',*,*,#16199,.F.);
#22098=ORIENTED_EDGE('',*,*,#16194,.F.);
#22099=ORIENTED_EDGE('',*,*,#16191,.F.);
#22100=ORIENTED_EDGE('',*,*,#16190,.F.);
#28283=PLANE('',#31722);
#28284=PLANE('',#31725);
#28285=PLANE('',#31726);
#28286=PLANE('',#31727);
#28287=PLANE('',#31728);
#28288=PLANE('',#31729);
#28289=PLANE('',#31730);
#28290=PLANE('',#31731);
#28291=PLANE('',#31732);
#28292=PLANE('',#31733);
#28293=PLANE('',#31734);
#28294=PLANE('',#31737);
#28295=PLANE('',#31740);
#28296=PLANE('',#31741);
#28297=PLANE('',#31742);
#28298=PLANE('',#31743);
#28299=PLANE('',#31744);
#28300=PLANE('',#31745);
#28301=PLANE('',#31746);
#28302=PLANE('',#31747);
#28303=PLANE('',#31749);
#28304=PLANE('',#31751);
#28305=PLANE('',#31753);
#28306=PLANE('',#31760);
#28307=PLANE('',#31763);
#28308=PLANE('',#31765);
#29465=ADVANCED_FACE('',(#4137),#2029,.F.);
#29466=ADVANCED_FACE('',(#4138),#2030,.F.);
#29467=ADVANCED_FACE('',(#4139),#538,.F.);
#29468=ADVANCED_FACE('',(#4140),#28283,.T.);
#29469=ADVANCED_FACE('',(#4141),#539,.F.);
#29470=ADVANCED_FACE('',(#4142),#28284,.T.);
#29471=ADVANCED_FACE('',(#4143),#28285,.T.);
#29472=ADVANCED_FACE('',(#4144),#28286,.T.);
#29473=ADVANCED_FACE('',(#4145),#28287,.T.);
#29474=ADVANCED_FACE('',(#4146),#28288,.T.);
#29475=ADVANCED_FACE('',(#4147),#28289,.T.);
#29476=ADVANCED_FACE('',(#4148),#28290,.T.);
#29477=ADVANCED_FACE('',(#4149),#28291,.T.);
#29478=ADVANCED_FACE('',(#4150),#28292,.T.);
#29479=ADVANCED_FACE('',(#4151,#3434,#3435),#28293,.T.);
#29480=ADVANCED_FACE('',(#4152,#3436,#3437),#28294,.T.);
#29481=ADVANCED_FACE('',(#4153),#28295,.T.);
#29482=ADVANCED_FACE('',(#4154),#28296,.T.);
#29483=ADVANCED_FACE('',(#4155),#28297,.F.);
#29484=ADVANCED_FACE('',(#4156),#28298,.T.);
#29485=ADVANCED_FACE('',(#4157),#28299,.T.);
#29486=ADVANCED_FACE('',(#4158),#28300,.T.);
#29487=ADVANCED_FACE('',(#4159),#28301,.T.);
#29488=ADVANCED_FACE('',(#4160,#3438),#28302,.T.);
#29489=ADVANCED_FACE('',(#4161,#3439),#28303,.T.);
#29490=ADVANCED_FACE('',(#4162,#3440),#28304,.F.);
#29491=ADVANCED_FACE('',(#4163,#3441),#28305,.F.);
#29492=ADVANCED_FACE('',(#4164),#540,.F.);
#29493=ADVANCED_FACE('',(#4165),#541,.F.);
#29494=ADVANCED_FACE('',(#4166),#542,.F.);
#29495=ADVANCED_FACE('',(#4167),#543,.F.);
#29496=ADVANCED_FACE('',(#4168),#28306,.T.);
#29497=ADVANCED_FACE('',(#4169,#3442),#544,.F.);
#29498=ADVANCED_FACE('',(#4170),#28307,.F.);
#29499=ADVANCED_FACE('',(#4171),#545,.F.);
#29500=ADVANCED_FACE('',(#4172),#28308,.T.);
#30664=CLOSED_SHELL('',(#29465,#29466,#29467,#29468,#29469,#29470,#29471,
#29472,#29473,#29474,#29475,#29476,#29477,#29478,#29479,#29480,#29481,#29482,
#29483,#29484,#29485,#29486,#29487,#29488,#29489,#29490,#29491,#29492,#29493,
#29494,#29495,#29496,#29497,#29498,#29499,#29500));
#31710=AXIS2_PLACEMENT_3D('',#44566,#35783,#35784);
#31711=AXIS2_PLACEMENT_3D('',#44567,#35785,#35786);
#31712=AXIS2_PLACEMENT_3D('',#44577,#35787,#35788);
#31713=AXIS2_PLACEMENT_3D('',#44580,#35790,#35791);
#31714=AXIS2_PLACEMENT_3D('',#44581,#35792,#35793);
#31715=AXIS2_PLACEMENT_3D('',#44582,#35794,#35795);
#31716=AXIS2_PLACEMENT_3D('',#44584,#35796,#35797);
#31717=AXIS2_PLACEMENT_3D('',#44587,#35799,#35800);
#31718=AXIS2_PLACEMENT_3D('',#44589,#35801,#35802);
#31719=AXIS2_PLACEMENT_3D('',#44594,#35803,#35804);
#31720=AXIS2_PLACEMENT_3D('',#44595,#35805,#35806);
#31721=AXIS2_PLACEMENT_3D('',#44598,#35808,#35809);
#31722=AXIS2_PLACEMENT_3D('',#44599,#35810,#35811);
#31723=AXIS2_PLACEMENT_3D('',#44611,#35818,#35819);
#31724=AXIS2_PLACEMENT_3D('',#44614,#35821,#35822);
#31725=AXIS2_PLACEMENT_3D('',#44615,#35823,#35824);
#31726=AXIS2_PLACEMENT_3D('',#44619,#35827,#35828);
#31727=AXIS2_PLACEMENT_3D('',#44626,#35832,#35833);
#31728=AXIS2_PLACEMENT_3D('',#44629,#35836,#35837);
#31729=AXIS2_PLACEMENT_3D('',#44637,#35842,#35843);
#31730=AXIS2_PLACEMENT_3D('',#44644,#35847,#35848);
#31731=AXIS2_PLACEMENT_3D('',#44649,#35852,#35853);
#31732=AXIS2_PLACEMENT_3D('',#44652,#35856,#35857);
#31733=AXIS2_PLACEMENT_3D('',#44660,#35862,#35863);
#31734=AXIS2_PLACEMENT_3D('',#44668,#35868,#35869);
#31735=AXIS2_PLACEMENT_3D('',#44671,#35871,#35872);
#31736=AXIS2_PLACEMENT_3D('',#44673,#35873,#35874);
#31737=AXIS2_PLACEMENT_3D('',#44674,#35875,#35876);
#31738=AXIS2_PLACEMENT_3D('',#44677,#35878,#35879);
#31739=AXIS2_PLACEMENT_3D('',#44679,#35880,#35881);
#31740=AXIS2_PLACEMENT_3D('',#44680,#35882,#35883);
#31741=AXIS2_PLACEMENT_3D('',#44686,#35887,#35888);
#31742=AXIS2_PLACEMENT_3D('',#44692,#35892,#35893);
#31743=AXIS2_PLACEMENT_3D('',#44693,#35894,#35895);
#31744=AXIS2_PLACEMENT_3D('',#44697,#35898,#35899);
#31745=AXIS2_PLACEMENT_3D('',#44700,#35902,#35903);
#31746=AXIS2_PLACEMENT_3D('',#44704,#35906,#35907);
#31747=AXIS2_PLACEMENT_3D('',#44707,#35910,#35911);
#31748=AXIS2_PLACEMENT_3D('',#44709,#35912,#35913);
#31749=AXIS2_PLACEMENT_3D('',#44710,#35914,#35915);
#31750=AXIS2_PLACEMENT_3D('',#44712,#35916,#35917);
#31751=AXIS2_PLACEMENT_3D('',#44713,#35918,#35919);
#31752=AXIS2_PLACEMENT_3D('',#44715,#35920,#35921);
#31753=AXIS2_PLACEMENT_3D('',#44716,#35922,#35923);
#31754=AXIS2_PLACEMENT_3D('',#44718,#35924,#35925);
#31755=AXIS2_PLACEMENT_3D('',#44719,#35926,#35927);
#31756=AXIS2_PLACEMENT_3D('',#44721,#35929,#35930);
#31757=AXIS2_PLACEMENT_3D('',#44723,#35932,#35933);
#31758=AXIS2_PLACEMENT_3D('',#44766,#35935,#35936);
#31759=AXIS2_PLACEMENT_3D('',#44807,#35938,#35939);
#31760=AXIS2_PLACEMENT_3D('',#44808,#35940,#35941);
#31761=AXIS2_PLACEMENT_3D('',#44809,#35942,#35943);
#31762=AXIS2_PLACEMENT_3D('',#44813,#35946,#35947);
#31763=AXIS2_PLACEMENT_3D('',#44814,#35948,#35949);
#31764=AXIS2_PLACEMENT_3D('',#44815,#35950,#35951);
#31765=AXIS2_PLACEMENT_3D('',#44817,#35953,#35954);
#35783=DIRECTION('axis',(0.,0.,1.));
#35784=DIRECTION('refdir',(1.,0.,0.));
#35785=DIRECTION('center_axis',(0.,-1.,0.));
#35786=DIRECTION('ref_axis',(1.,0.,0.));
#35787=DIRECTION('center_axis',(0.,-1.,0.));
#35788=DIRECTION('ref_axis',(1.,0.,0.));
#35789=DIRECTION('',(0.707106781186543,0.707106781186552,8.65956056235487E-17));
#35790=DIRECTION('center_axis',(0.,1.,0.));
#35791=DIRECTION('ref_axis',(1.,0.,0.));
#35792=DIRECTION('center_axis',(0.,-1.,0.));
#35793=DIRECTION('ref_axis',(1.,0.,0.));
#35794=DIRECTION('center_axis',(0.,-1.,0.));
#35795=DIRECTION('ref_axis',(1.,0.,0.));
#35796=DIRECTION('center_axis',(0.,-1.,0.));
#35797=DIRECTION('ref_axis',(1.,0.,0.));
#35798=DIRECTION('',(0.707106781186543,0.707106781186552,8.65956056235487E-17));
#35799=DIRECTION('center_axis',(0.,1.,0.));
#35800=DIRECTION('ref_axis',(1.,0.,0.));
#35801=DIRECTION('center_axis',(0.,-1.,0.));
#35802=DIRECTION('ref_axis',(1.,0.,0.));
#35803=DIRECTION('center_axis',(0.,-1.,0.));
#35804=DIRECTION('ref_axis',(1.,0.,0.));
#35805=DIRECTION('center_axis',(0.,1.,0.));
#35806=DIRECTION('ref_axis',(1.,0.,0.));
#35807=DIRECTION('',(0.,1.,0.));
#35808=DIRECTION('center_axis',(0.,1.,0.));
#35809=DIRECTION('ref_axis',(1.,0.,0.));
#35810=DIRECTION('center_axis',(0.,-0.707106781186543,-0.707106781186553));
#35811=DIRECTION('ref_axis',(-1.,0.,0.));
#35812=DIRECTION('',(-1.,0.,0.));
#35813=DIRECTION('',(-1.25607396694701E-14,0.707106781186552,-0.707106781186542));
#35814=DIRECTION('',(1.,0.,0.));
#35815=DIRECTION('',(-0.577350269189618,0.577350269189634,-0.577350269189625));
#35816=DIRECTION('',(-0.577350269189622,-0.577350269189632,0.577350269189624));
#35817=DIRECTION('',(-1.,0.,0.));
#35818=DIRECTION('center_axis',(0.,1.,0.));
#35819=DIRECTION('ref_axis',(1.,0.,0.));
#35820=DIRECTION('',(0.,1.,0.));
#35821=DIRECTION('center_axis',(0.,1.,0.));
#35822=DIRECTION('ref_axis',(1.,0.,0.));
#35823=DIRECTION('center_axis',(-0.577350269189627,-0.577350269189626,-0.577350269189624));
#35824=DIRECTION('ref_axis',(-0.707106781186546,0.,0.707106781186549));
#35825=DIRECTION('',(0.707106781186547,-0.707106781186547,0.));
#35826=DIRECTION('',(-0.707106781186546,0.,0.707106781186549));
#35827=DIRECTION('center_axis',(-0.577350269189627,0.577350269189627,-0.577350269189624));
#35828=DIRECTION('ref_axis',(-0.707106781186546,0.,0.707106781186549));
#35829=DIRECTION('',(0.,0.707106781186546,0.707106781186549));
#35830=DIRECTION('',(0.707106781186546,0.,-0.707106781186549));
#35831=DIRECTION('',(-0.707106781186548,-0.707106781186548,0.));
#35832=DIRECTION('center_axis',(-0.707106781186549,0.,-0.707106781186546));
#35833=DIRECTION('ref_axis',(-0.707106781186546,0.,0.707106781186549));
#35834=DIRECTION('',(0.,1.,0.));
#35835=DIRECTION('',(0.,-1.,0.));
#35836=DIRECTION('center_axis',(-0.707106781186548,0.707106781186548,0.));
#35837=DIRECTION('ref_axis',(0.,0.,1.));
#35838=DIRECTION('',(0.577350269189626,0.577350269189626,-0.577350269189626));
#35839=DIRECTION('',(0.,0.,-1.));
#35840=DIRECTION('',(0.,0.,1.));
#35841=DIRECTION('',(0.577350269189626,0.577350269189626,0.577350269189626));
#35842=DIRECTION('center_axis',(0.577350269189628,0.577350269189628,-0.577350269189621));
#35843=DIRECTION('ref_axis',(-0.707106781186543,0.,-0.707106781186552));
#35844=DIRECTION('',(-0.707106781186548,0.707106781186548,0.));
#35845=DIRECTION('',(0.707106781186543,0.,0.707106781186552));
#35846=DIRECTION('',(6.28036983473511E-15,-0.707106781186546,-0.707106781186549));
#35847=DIRECTION('center_axis',(0.707106781186552,0.,-0.707106781186543));
#35848=DIRECTION('ref_axis',(-0.707106781186543,0.,-0.707106781186552));
#35849=DIRECTION('',(0.,1.,0.));
#35850=DIRECTION('',(0.,-1.,0.));
#35851=DIRECTION('',(-0.57735026918962,-0.57735026918963,-0.577350269189627));
#35852=DIRECTION('center_axis',(0.,0.707106781186549,-0.707106781186546));
#35853=DIRECTION('ref_axis',(-1.,0.,0.));
#35854=DIRECTION('',(1.,0.,0.));
#35855=DIRECTION('',(-1.,0.,0.));
#35856=DIRECTION('center_axis',(0.707106781186548,0.707106781186548,0.));
#35857=DIRECTION('ref_axis',(0.,0.,-1.));
#35858=DIRECTION('',(0.577350269189626,-0.577350269189626,-0.577350269189626));
#35859=DIRECTION('',(0.,0.,-1.));
#35860=DIRECTION('',(0.,0.,1.));
#35861=DIRECTION('',(0.577350269189626,-0.577350269189626,0.577350269189626));
#35862=DIRECTION('center_axis',(-0.707106781186548,-0.707106781186548,0.));
#35863=DIRECTION('ref_axis',(0.,0.,1.));
#35864=DIRECTION('',(-0.577350269189626,0.577350269189626,-0.577350269189626));
#35865=DIRECTION('',(0.,0.,-1.));
#35866=DIRECTION('',(0.,0.,1.));
#35867=DIRECTION('',(-0.577350269189629,0.577350269189629,0.577350269189619));
#35868=DIRECTION('center_axis',(0.,1.,0.));
#35869=DIRECTION('ref_axis',(-1.,0.,0.));
#35870=DIRECTION('',(-1.,0.,0.));
#35871=DIRECTION('center_axis',(0.,-1.,0.));
#35872=DIRECTION('ref_axis',(1.,0.,0.));
#35873=DIRECTION('center_axis',(0.,-1.,0.));
#35874=DIRECTION('ref_axis',(1.,0.,0.));
#35875=DIRECTION('center_axis',(-1.,0.,0.));
#35876=DIRECTION('ref_axis',(0.,-1.,0.));
#35877=DIRECTION('',(0.,-1.,0.));
#35878=DIRECTION('center_axis',(1.,0.,0.));
#35879=DIRECTION('ref_axis',(0.,0.,-1.));
#35880=DIRECTION('center_axis',(1.,0.,0.));
#35881=DIRECTION('ref_axis',(0.,0.,-1.));
#35882=DIRECTION('center_axis',(-0.707106781186548,0.,0.707106781186548));
#35883=DIRECTION('ref_axis',(0.707106781186548,0.,0.707106781186548));
#35884=DIRECTION('',(-0.577350269189622,-0.577350269189633,-0.577350269189622));
#35885=DIRECTION('',(0.,1.,0.));
#35886=DIRECTION('',(-0.577350269189626,0.577350269189626,-0.577350269189626));
#35887=DIRECTION('center_axis',(0.,-0.707106781186541,0.707106781186554));
#35888=DIRECTION('ref_axis',(1.,0.,0.));
#35889=DIRECTION('',(1.,0.,0.));
#35890=DIRECTION('',(0.,0.707106781186554,0.707106781186541));
#35891=DIRECTION('',(-1.,0.,0.));
#35892=DIRECTION('center_axis',(0.,0.,1.));
#35893=DIRECTION('ref_axis',(1.,0.,0.));
#35894=DIRECTION('center_axis',(0.577350269189629,-0.577350269189619,0.577350269189629));
#35895=DIRECTION('ref_axis',(0.707106781186548,0.,-0.707106781186548));
#35896=DIRECTION('',(-0.707106781186541,-0.707106781186554,0.));
#35897=DIRECTION('',(0.707106781186548,0.,-0.707106781186548));
#35898=DIRECTION('center_axis',(0.707106781186554,-0.707106781186541,0.));
#35899=DIRECTION('ref_axis',(0.,0.,-1.));
#35900=DIRECTION('',(0.,0.,1.));
#35901=DIRECTION('',(0.,0.,-1.));
#35902=DIRECTION('center_axis',(0.,0.707106781186548,0.707106781186548));
#35903=DIRECTION('ref_axis',(1.,0.,0.));
#35904=DIRECTION('',(1.,0.,0.));
#35905=DIRECTION('',(0.577350269189626,0.577350269189626,-0.577350269189626));
#35906=DIRECTION('center_axis',(0.707106781186548,0.,0.707106781186548));
#35907=DIRECTION('ref_axis',(0.707106781186548,0.,-0.707106781186548));
#35908=DIRECTION('',(0.,-1.,0.));
#35909=DIRECTION('',(0.,1.,0.));
#35910=DIRECTION('center_axis',(1.,0.,0.));
#35911=DIRECTION('ref_axis',(0.,1.,0.));
#35912=DIRECTION('center_axis',(-1.,0.,0.));
#35913=DIRECTION('ref_axis',(0.,0.,-1.));
#35914=DIRECTION('center_axis',(0.,0.,1.));
#35915=DIRECTION('ref_axis',(1.,0.,0.));
#35916=DIRECTION('center_axis',(0.,0.,-1.));
#35917=DIRECTION('ref_axis',(1.,0.,0.));
#35918=DIRECTION('center_axis',(0.,1.,0.));
#35919=DIRECTION('ref_axis',(1.,0.,0.));
#35920=DIRECTION('center_axis',(0.,-1.,0.));
#35921=DIRECTION('ref_axis',(1.,0.,0.));
#35922=DIRECTION('center_axis',(0.,1.,0.));
#35923=DIRECTION('ref_axis',(1.,0.,0.));
#35924=DIRECTION('center_axis',(0.,-1.,0.));
#35925=DIRECTION('ref_axis',(1.,0.,0.));
#35926=DIRECTION('center_axis',(0.,1.,0.));
#35927=DIRECTION('ref_axis',(1.,0.,0.));
#35928=DIRECTION('',(0.,1.,0.));
#35929=DIRECTION('center_axis',(0.,1.,0.));
#35930=DIRECTION('ref_axis',(1.,0.,0.));
#35931=DIRECTION('',(0.,1.,0.));
#35932=DIRECTION('center_axis',(0.,0.,-1.));
#35933=DIRECTION('ref_axis',(1.,0.,0.));
#35934=DIRECTION('',(0.,0.,-1.));
#35935=DIRECTION('center_axis',(0.,0.,-1.));
#35936=DIRECTION('ref_axis',(1.,0.,0.));
#35937=DIRECTION('',(0.,0.,-1.));
#35938=DIRECTION('center_axis',(0.,0.,-1.));
#35939=DIRECTION('ref_axis',(1.,0.,0.));
#35940=DIRECTION('center_axis',(0.,0.,1.));
#35941=DIRECTION('ref_axis',(1.,0.,0.));
#35942=DIRECTION('center_axis',(1.,0.,0.));
#35943=DIRECTION('ref_axis',(0.,0.,-1.));
#35944=DIRECTION('',(1.,0.,0.));
#35945=DIRECTION('',(1.,0.,0.));
#35946=DIRECTION('center_axis',(1.,0.,0.));
#35947=DIRECTION('ref_axis',(0.,0.,-1.));
#35948=DIRECTION('center_axis',(1.,0.,0.));
#35949=DIRECTION('ref_axis',(0.,0.,-1.));
#35950=DIRECTION('center_axis',(-1.,0.,0.));
#35951=DIRECTION('ref_axis',(0.,0.,-1.));
#35952=DIRECTION('',(-1.,0.,0.));
#35953=DIRECTION('center_axis',(0.,-1.,0.));
#35954=DIRECTION('ref_axis',(1.,0.,0.));
#44566=CARTESIAN_POINT('',(0.,0.,0.));
#44567=CARTESIAN_POINT('Origin',(-33.475,-85.475,10.75));
#44568=CARTESIAN_POINT('',(-34.8212912017836,-85.725,7.25));
#44569=CARTESIAN_POINT('',(-32.1287087982164,-85.725,7.25));
#44570=CARTESIAN_POINT('Ctrl Pts',(-34.8212912017836,-85.725,7.25));
#44571=CARTESIAN_POINT('Ctrl Pts',(-34.4096238271454,-85.5772068894569,
7.25));
#44572=CARTESIAN_POINT('Ctrl Pts',(-33.9716586462892,-85.475,7.25));
#44573=CARTESIAN_POINT('Ctrl Pts',(-32.9783413537108,-85.475,7.25));
#44574=CARTESIAN_POINT('Ctrl Pts',(-32.5403761728546,-85.5772068894569,
7.25));
#44575=CARTESIAN_POINT('Ctrl Pts',(-32.1287087982164,-85.725,7.25));
#44576=CARTESIAN_POINT('',(-37.225,-85.725,10.75));
#44577=CARTESIAN_POINT('Origin',(-33.475,-85.725,10.75));
#44578=CARTESIAN_POINT('',(-36.725,-85.225,10.75));
#44579=CARTESIAN_POINT('',(-36.975,-85.475,10.75));
#44580=CARTESIAN_POINT('Origin',(-33.475,-85.225,10.75));
#44581=CARTESIAN_POINT('Origin',(-33.475,-85.725,10.75));
#44582=CARTESIAN_POINT('Origin',(-33.475,-85.475,3.75));
#44583=CARTESIAN_POINT('',(-37.225,-85.725,3.75));
#44584=CARTESIAN_POINT('Origin',(-33.475,-85.725,3.75));
#44585=CARTESIAN_POINT('',(-36.725,-85.225,3.75));
#44586=CARTESIAN_POINT('',(-36.975,-85.475,3.75));
#44587=CARTESIAN_POINT('Origin',(-33.475,-85.225,3.75));
#44588=CARTESIAN_POINT('',(-35.345828693387,-85.725,0.5));
#44589=CARTESIAN_POINT('Origin',(-33.475,-85.725,3.75));
#44590=CARTESIAN_POINT('',(-31.604171306613,-85.725,0.5));
#44591=CARTESIAN_POINT('Ctrl Pts',(-35.345828693387,-85.725,0.500000000000002));
#44592=CARTESIAN_POINT('Ctrl Pts',(-33.475,-85.225,-9.0205620750794E-16));
#44593=CARTESIAN_POINT('Ctrl Pts',(-31.604171306613,-85.725,0.500000000000002));
#44594=CARTESIAN_POINT('Origin',(-33.475,-85.725,3.75));
#44595=CARTESIAN_POINT('Origin',(-33.475,-85.725,10.75));
#44596=CARTESIAN_POINT('',(-36.725,-73.225,10.75));
#44597=CARTESIAN_POINT('',(-36.725,-85.725,10.75));
#44598=CARTESIAN_POINT('Origin',(-33.475,-73.225,10.75));
#44599=CARTESIAN_POINT('Origin',(-37.05,-85.475,0.25));
#44600=CARTESIAN_POINT('',(-40.125,-85.725,0.5));
#44601=CARTESIAN_POINT('',(-37.05,-85.725,0.5));
#44602=CARTESIAN_POINT('',(-40.125,-85.225,0.));
#44603=CARTESIAN_POINT('',(-40.125,-85.725,0.5));
#44604=CARTESIAN_POINT('',(-26.825,-85.225,0.));
#44605=CARTESIAN_POINT('',(-37.05,-85.225,0.));
#44606=CARTESIAN_POINT('',(-26.575,-85.475,0.250000000000002));
#44607=CARTESIAN_POINT('',(-29.9041666666666,-82.1458333333333,-3.07916666666666));
#44608=CARTESIAN_POINT('',(-26.825,-85.725,0.5));
#44609=CARTESIAN_POINT('',(-28.2791666666666,-87.1791666666667,1.95416666666665));
#44610=CARTESIAN_POINT('',(-37.05,-85.725,0.5));
#44611=CARTESIAN_POINT('Origin',(-33.475,-85.725,3.75));
#44612=CARTESIAN_POINT('',(-36.725,-73.225,3.75));
#44613=CARTESIAN_POINT('',(-36.725,-85.725,3.75));
#44614=CARTESIAN_POINT('Origin',(-33.475,-73.225,3.75));
#44615=CARTESIAN_POINT('Origin',(-40.125,-85.225,0.));
#44616=CARTESIAN_POINT('',(-40.625,-85.225,0.5));
#44617=CARTESIAN_POINT('',(-40.625,-85.225,0.5));
#44618=CARTESIAN_POINT('',(-40.125,-85.225,0.));
#44619=CARTESIAN_POINT('Origin',(-40.625,-47.225,0.5));
#44620=CARTESIAN_POINT('',(-40.125,-47.225,0.));
#44621=CARTESIAN_POINT('',(-40.125,-46.725,0.5));
#44622=CARTESIAN_POINT('',(-40.125,-47.225,0.));
#44623=CARTESIAN_POINT('',(-40.625,-47.225,0.5));
#44624=CARTESIAN_POINT('',(-40.625,-47.225,0.5));
#44625=CARTESIAN_POINT('',(-40.125,-46.725,0.5));
#44626=CARTESIAN_POINT('Origin',(-40.375,-56.475,0.25));
#44627=CARTESIAN_POINT('',(-40.625,-56.475,0.5));
#44628=CARTESIAN_POINT('',(-40.125,-56.475,0.));
#44629=CARTESIAN_POINT('Origin',(-40.375,-46.975,0.));
#44630=CARTESIAN_POINT('',(-40.375,-46.975,31.75));
#44631=CARTESIAN_POINT('',(-40.125,-46.725,31.5));
#44632=CARTESIAN_POINT('',(-33.3375,-39.9375,24.7125));
#44633=CARTESIAN_POINT('',(-40.125,-46.725,0.));
#44634=CARTESIAN_POINT('',(-40.625,-47.225,31.5));
#44635=CARTESIAN_POINT('',(-40.625,-47.225,0.));
#44636=CARTESIAN_POINT('',(-47.25,-53.85,24.875));
#44637=CARTESIAN_POINT('Origin',(-26.825,-47.225,0.));
#44638=CARTESIAN_POINT('',(-26.325,-47.225,0.5));
#44639=CARTESIAN_POINT('',(-26.825,-46.725,0.5));
#44640=CARTESIAN_POINT('',(-26.325,-47.225,0.5));
#44641=CARTESIAN_POINT('',(-26.825,-47.225,0.));
#44642=CARTESIAN_POINT('',(-26.825,-47.225,0.));
#44643=CARTESIAN_POINT('',(-26.825,-46.725,0.5));
#44644=CARTESIAN_POINT('Origin',(-26.575,-75.975,0.25));
#44645=CARTESIAN_POINT('',(-26.825,-75.975,0.));
#44646=CARTESIAN_POINT('',(-26.325,-85.225,0.5));
#44647=CARTESIAN_POINT('',(-26.325,-75.975,0.5));
#44648=CARTESIAN_POINT('',(-25.0333333333333,-83.9333333333333,1.79166666666668));
#44649=CARTESIAN_POINT('Origin',(-29.9,-46.975,0.25));
#44650=CARTESIAN_POINT('',(-29.9,-46.725,0.5));
#44651=CARTESIAN_POINT('',(-29.9,-47.225,0.));
#44652=CARTESIAN_POINT('Origin',(-26.575,-46.975,0.));
#44653=CARTESIAN_POINT('',(-26.575,-46.975,31.75));
#44654=CARTESIAN_POINT('',(-26.325,-47.225,31.5));
#44655=CARTESIAN_POINT('',(-16.45,-57.1,21.625));
#44656=CARTESIAN_POINT('',(-26.325,-47.225,0.));
#44657=CARTESIAN_POINT('',(-26.825,-46.725,31.5));
#44658=CARTESIAN_POINT('',(-26.825,-46.725,0.));
#44659=CARTESIAN_POINT('',(-32.4208333333333,-41.1291666666667,25.9041666666667));
#44660=CARTESIAN_POINT('Origin',(-40.375,-85.475,0.));
#44661=CARTESIAN_POINT('',(-40.375,-85.475,31.75));
#44662=CARTESIAN_POINT('',(-40.625,-85.225,31.5));
#44663=CARTESIAN_POINT('',(-50.5,-75.35,21.625));
#44664=CARTESIAN_POINT('',(-40.625,-85.225,0.));
#44665=CARTESIAN_POINT('',(-40.125,-85.725,31.5));
#44666=CARTESIAN_POINT('',(-40.125,-85.725,0.));
#44667=CARTESIAN_POINT('',(-34.5291666666667,-91.3208333333333,25.9041666666668));
#44668=CARTESIAN_POINT('Origin',(-26.325,-46.725,0.));
#44669=CARTESIAN_POINT('',(-29.9,-46.725,31.5));
#44670=CARTESIAN_POINT('',(-35.175,-46.725,10.75));
#44671=CARTESIAN_POINT('Origin',(-33.475,-46.725,10.75));
#44672=CARTESIAN_POINT('',(-35.175,-46.725,3.75));
#44673=CARTESIAN_POINT('Origin',(-33.475,-46.725,3.75));
#44674=CARTESIAN_POINT('Origin',(-40.625,-46.725,0.));
#44675=CARTESIAN_POINT('',(-40.625,-56.475,31.5));
#44676=CARTESIAN_POINT('',(-40.625,-66.,27.05));
#44677=CARTESIAN_POINT('Origin',(-40.625,-66.,20.));
#44678=CARTESIAN_POINT('',(-40.625,-79.,24.5));
#44679=CARTESIAN_POINT('Origin',(-40.625,-79.,20.));
#44680=CARTESIAN_POINT('Origin',(-40.375,-56.475,31.75));
#44681=CARTESIAN_POINT('',(-40.125,-85.225,32.));
#44682=CARTESIAN_POINT('',(-40.125,-85.225,32.));
#44683=CARTESIAN_POINT('',(-40.125,-47.225,32.));
#44684=CARTESIAN_POINT('',(-40.125,-56.475,32.));
#44685=CARTESIAN_POINT('',(-40.125,-47.225,32.));
#44686=CARTESIAN_POINT('Origin',(-37.05,-85.475,31.75));
#44687=CARTESIAN_POINT('',(-26.825,-85.725,31.5));
#44688=CARTESIAN_POINT('',(-37.05,-85.725,31.5));
#44689=CARTESIAN_POINT('',(-26.825,-85.225,32.));
#44690=CARTESIAN_POINT('',(-26.825,-85.725,31.5));
#44691=CARTESIAN_POINT('',(-37.05,-85.225,32.));
#44692=CARTESIAN_POINT('Origin',(-33.475,-66.225,0.));
#44693=CARTESIAN_POINT('Origin',(-26.325,-85.225,31.5));
#44694=CARTESIAN_POINT('',(-26.325,-85.225,31.5));
#44695=CARTESIAN_POINT('',(-26.325,-85.225,31.5));
#44696=CARTESIAN_POINT('',(-26.825,-85.225,32.));
#44697=CARTESIAN_POINT('Origin',(-26.575,-85.475,0.));
#44698=CARTESIAN_POINT('',(-26.325,-85.225,0.));
#44699=CARTESIAN_POINT('',(-26.825,-85.725,0.));
#44700=CARTESIAN_POINT('Origin',(-29.9,-46.975,31.75));
#44701=CARTESIAN_POINT('',(-26.825,-47.225,32.));
#44702=CARTESIAN_POINT('',(-29.9,-47.225,32.));
#44703=CARTESIAN_POINT('',(-26.825,-47.225,32.));
#44704=CARTESIAN_POINT('Origin',(-26.575,-75.975,31.75));
#44705=CARTESIAN_POINT('',(-26.825,-75.975,32.));
#44706=CARTESIAN_POINT('',(-26.325,-75.975,31.5));
#44707=CARTESIAN_POINT('Origin',(-26.325,-85.725,0.));
#44708=CARTESIAN_POINT('',(-26.325,-66.,27.05));
#44709=CARTESIAN_POINT('Origin',(-26.325,-66.,20.));
#44710=CARTESIAN_POINT('Origin',(-33.475,-66.225,32.));
#44711=CARTESIAN_POINT('',(-40.1,-79.,32.));
#44712=CARTESIAN_POINT('Origin',(-38.6,-79.,32.));
#44713=CARTESIAN_POINT('Origin',(-33.475,-73.225,3.75));
#44714=CARTESIAN_POINT('',(-35.175,-73.225,3.75));
#44715=CARTESIAN_POINT('Origin',(-33.475,-73.225,3.75));
#44716=CARTESIAN_POINT('Origin',(-33.475,-73.225,10.75));
#44717=CARTESIAN_POINT('',(-35.175,-73.225,10.75));
#44718=CARTESIAN_POINT('Origin',(-33.475,-73.225,10.75));
#44719=CARTESIAN_POINT('Origin',(-33.475,-85.725,3.75));
#44720=CARTESIAN_POINT('',(-35.175,-85.725,3.75));
#44721=CARTESIAN_POINT('Origin',(-33.475,-85.725,10.75));
#44722=CARTESIAN_POINT('',(-35.175,-85.725,10.75));
#44723=CARTESIAN_POINT('Origin',(-38.6,-79.,32.));
#44724=CARTESIAN_POINT('',(-40.1,-79.,24.5));
#44725=CARTESIAN_POINT('',(-40.1,-79.,32.));
#44726=CARTESIAN_POINT('',(-38.6,-77.5,24.2426406871193));
#44727=CARTESIAN_POINT('Ctrl Pts',(-38.6,-77.5,24.2426406871193));
#44728=CARTESIAN_POINT('Ctrl Pts',(-38.7899690906118,-77.5,24.2426406871193));
#44729=CARTESIAN_POINT('Ctrl Pts',(-38.9915029601953,-77.5382644910968,
24.2567401743069));
#44730=CARTESIAN_POINT('Ctrl Pts',(-39.3605797699365,-77.6917706385605,
24.3063956191435));
#44731=CARTESIAN_POINT('Ctrl Pts',(-39.5282646235601,-77.8069442800005,
24.3411032840945));
#44732=CARTESIAN_POINT('Ctrl Pts',(-39.7929943148421,-78.0716739712825,
24.4053096652352));
#44733=CARTESIAN_POINT('Ctrl Pts',(-39.9082152291749,-78.2393832820639,
24.4391554329551));
#44734=CARTESIAN_POINT('Ctrl Pts',(-40.0617566312046,-78.6085507941687,
24.4868035691518));
#44735=CARTESIAN_POINT('Ctrl Pts',(-40.1,-78.810119017199,24.5));
#44736=CARTESIAN_POINT('Ctrl Pts',(-40.1,-79.,24.5));
#44737=CARTESIAN_POINT('',(-37.1,-79.,24.5));
#44738=CARTESIAN_POINT('Ctrl Pts',(-37.1,-79.,24.5));
#44739=CARTESIAN_POINT('Ctrl Pts',(-37.1,-78.810119017199,24.5));
#44740=CARTESIAN_POINT('Ctrl Pts',(-37.1382433687954,-78.6085507941687,
24.4868035691518));
#44741=CARTESIAN_POINT('Ctrl Pts',(-37.2917847708251,-78.2393832820639,
24.4391554329551));
#44742=CARTESIAN_POINT('Ctrl Pts',(-37.4070056851579,-78.0716739712825,
24.4053096652352));
#44743=CARTESIAN_POINT('Ctrl Pts',(-37.6717353764399,-77.8069442800005,
24.3411032840945));
#44744=CARTESIAN_POINT('Ctrl Pts',(-37.8394202300635,-77.6917706385605,
24.3063956191435));
#44745=CARTESIAN_POINT('Ctrl Pts',(-38.2084970398047,-77.5382644910968,
24.2567401743069));
#44746=CARTESIAN_POINT('Ctrl Pts',(-38.4100309093882,-77.5,24.2426406871193));
#44747=CARTESIAN_POINT('Ctrl Pts',(-38.6,-77.5,24.2426406871193));
#44748=CARTESIAN_POINT('Ctrl Pts',(-40.1,-79.,24.5));
#44749=CARTESIAN_POINT('Ctrl Pts',(-40.1,-79.189880982801,24.5));
#44750=CARTESIAN_POINT('Ctrl Pts',(-40.0617566312046,-79.3914492058313,
24.4868035691518));
#44751=CARTESIAN_POINT('Ctrl Pts',(-39.9082152291749,-79.7606167179361,
24.4391554329551));
#44752=CARTESIAN_POINT('Ctrl Pts',(-39.7929943148421,-79.9283260287175,
24.4053096652352));
#44753=CARTESIAN_POINT('Ctrl Pts',(-39.5282646235601,-80.1930557199996,
24.3411032840945));
#44754=CARTESIAN_POINT('Ctrl Pts',(-39.3605797699365,-80.3082293614395,
24.3063956191435));
#44755=CARTESIAN_POINT('Ctrl Pts',(-38.9915029601953,-80.4617355089032,
24.2567401743069));
#44756=CARTESIAN_POINT('Ctrl Pts',(-38.7899690906118,-80.5,24.2426406871193));
#44757=CARTESIAN_POINT('Ctrl Pts',(-38.4100309093882,-80.5,24.2426406871193));
#44758=CARTESIAN_POINT('Ctrl Pts',(-38.2084970398047,-80.4617355089032,
24.2567401743069));
#44759=CARTESIAN_POINT('Ctrl Pts',(-37.8394202300634,-80.3082293614395,
24.3063956191435));
#44760=CARTESIAN_POINT('Ctrl Pts',(-37.6717353764399,-80.1930557199996,
24.3411032840945));
#44761=CARTESIAN_POINT('Ctrl Pts',(-37.4070056851579,-79.9283260287175,
24.4053096652352));
#44762=CARTESIAN_POINT('Ctrl Pts',(-37.2917847708251,-79.7606167179361,
24.4391554329551));
#44763=CARTESIAN_POINT('Ctrl Pts',(-37.1382433687954,-79.3914492058313,
24.4868035691518));
#44764=CARTESIAN_POINT('Ctrl Pts',(-37.1,-79.189880982801,24.5));
#44765=CARTESIAN_POINT('Ctrl Pts',(-37.1,-79.,24.5));
#44766=CARTESIAN_POINT('Origin',(-38.6,-79.,32.));
#44767=CARTESIAN_POINT('',(-38.6,-77.5,15.7573593128807));
#44768=CARTESIAN_POINT('',(-40.1,-79.,15.5));
#44769=CARTESIAN_POINT('Ctrl Pts',(-38.6,-77.5,15.7573593128807));
#44770=CARTESIAN_POINT('Ctrl Pts',(-38.4100309093882,-77.5,15.7573593128807));
#44771=CARTESIAN_POINT('Ctrl Pts',(-38.2084970398047,-77.5382644910968,
15.7432598256931));
#44772=CARTESIAN_POINT('Ctrl Pts',(-37.8394202300635,-77.6917706385605,
15.6936043808565));
#44773=CARTESIAN_POINT('Ctrl Pts',(-37.6717353764399,-77.8069442800005,
15.6588967159055));
#44774=CARTESIAN_POINT('Ctrl Pts',(-37.4070056851579,-78.0716739712825,
15.5946903347648));
#44775=CARTESIAN_POINT('Ctrl Pts',(-37.2917847708251,-78.2393832820639,
15.5608445670449));
#44776=CARTESIAN_POINT('Ctrl Pts',(-37.1382433687954,-78.6085507941687,
15.5131964308482));
#44777=CARTESIAN_POINT('Ctrl Pts',(-37.1,-78.810119017199,15.5));
#44778=CARTESIAN_POINT('Ctrl Pts',(-37.1,-79.189880982801,15.5));
#44779=CARTESIAN_POINT('Ctrl Pts',(-37.1382433687954,-79.3914492058313,
15.5131964308482));
#44780=CARTESIAN_POINT('Ctrl Pts',(-37.2917847708251,-79.7606167179361,
15.5608445670449));
#44781=CARTESIAN_POINT('Ctrl Pts',(-37.4070056851579,-79.9283260287175,
15.5946903347648));
#44782=CARTESIAN_POINT('Ctrl Pts',(-37.6717353764399,-80.1930557199996,
15.6588967159055));
#44783=CARTESIAN_POINT('Ctrl Pts',(-37.8394202300635,-80.3082293614395,
15.6936043808565));
#44784=CARTESIAN_POINT('Ctrl Pts',(-38.2084970398047,-80.4617355089032,
15.7432598256931));
#44785=CARTESIAN_POINT('Ctrl Pts',(-38.4100309093882,-80.5,15.7573593128807));
#44786=CARTESIAN_POINT('Ctrl Pts',(-38.7899690906118,-80.5,15.7573593128807));
#44787=CARTESIAN_POINT('Ctrl Pts',(-38.9915029601953,-80.4617355089032,
15.7432598256931));
#44788=CARTESIAN_POINT('Ctrl Pts',(-39.3605797699366,-80.3082293614395,
15.6936043808565));
#44789=CARTESIAN_POINT('Ctrl Pts',(-39.5282646235601,-80.1930557199995,
15.6588967159055));
#44790=CARTESIAN_POINT('Ctrl Pts',(-39.7929943148421,-79.9283260287175,
15.5946903347648));
#44791=CARTESIAN_POINT('Ctrl Pts',(-39.9082152291749,-79.7606167179361,
15.5608445670449));
#44792=CARTESIAN_POINT('Ctrl Pts',(-40.0617566312046,-79.3914492058313,
15.5131964308482));
#44793=CARTESIAN_POINT('Ctrl Pts',(-40.1,-79.189880982801,15.5));
#44794=CARTESIAN_POINT('Ctrl Pts',(-40.1,-79.,15.5));
#44795=CARTESIAN_POINT('Ctrl Pts',(-40.1,-79.,15.5));
#44796=CARTESIAN_POINT('Ctrl Pts',(-40.1,-78.810119017199,15.5));
#44797=CARTESIAN_POINT('Ctrl Pts',(-40.0617566312046,-78.6085507941687,
15.5131964308482));
#44798=CARTESIAN_POINT('Ctrl Pts',(-39.9082152291749,-78.2393832820639,
15.5608445670449));
#44799=CARTESIAN_POINT('Ctrl Pts',(-39.7929943148421,-78.0716739712825,
15.5946903347648));
#44800=CARTESIAN_POINT('Ctrl Pts',(-39.5282646235601,-77.8069442800005,
15.6588967159055));
#44801=CARTESIAN_POINT('Ctrl Pts',(-39.3605797699365,-77.6917706385605,
15.6936043808565));
#44802=CARTESIAN_POINT('Ctrl Pts',(-38.9915029601953,-77.5382644910968,
15.7432598256931));
#44803=CARTESIAN_POINT('Ctrl Pts',(-38.7899690906118,-77.5,15.7573593128807));
#44804=CARTESIAN_POINT('Ctrl Pts',(-38.6,-77.5,15.7573593128807));
#44805=CARTESIAN_POINT('',(-40.1,-79.,14.));
#44806=CARTESIAN_POINT('',(-40.1,-79.,32.));
#44807=CARTESIAN_POINT('Origin',(-38.6,-79.,14.));
#44808=CARTESIAN_POINT('Origin',(-38.6,-79.,14.));
#44809=CARTESIAN_POINT('Origin',(-40.625,-79.,20.));
#44810=CARTESIAN_POINT('',(-40.625,-79.,24.5));
#44811=CARTESIAN_POINT('',(-30.625,-79.,24.5));
#44812=CARTESIAN_POINT('',(-40.625,-79.,24.5));
#44813=CARTESIAN_POINT('Origin',(-30.625,-79.,20.));
#44814=CARTESIAN_POINT('Origin',(-30.625,-79.,20.));
#44815=CARTESIAN_POINT('Origin',(-26.325,-66.,20.));
#44816=CARTESIAN_POINT('',(-26.325,-66.,27.05));
#44817=CARTESIAN_POINT('Origin',(-40.625,-85.725,0.));
#82347=UNCERTAINTY_MEASURE_WITH_UNIT(LENGTH_MEASURE(0.01),#82385,
'DISTANCE_ACCURACY_VALUE',
'Maximum model space distance between geometric entities at asserted c
onnectivities');
#82363=UNCERTAINTY_MEASURE_WITH_UNIT(LENGTH_MEASURE(0.01),#82385,
'DISTANCE_ACCURACY_VALUE',
'Maximum model space distance between geometric entities at asserted c
onnectivities');
#82368=(
GEOMETRIC_REPRESENTATION_CONTEXT(3)
GLOBAL_UNCERTAINTY_ASSIGNED_CONTEXT((#82347))
GLOBAL_UNIT_ASSIGNED_CONTEXT((#82385,#82387,#82388))
REPRESENTATION_CONTEXT('','3D')
);
#82384=(
GEOMETRIC_REPRESENTATION_CONTEXT(3)
GLOBAL_UNCERTAINTY_ASSIGNED_CONTEXT((#82363))
GLOBAL_UNIT_ASSIGNED_CONTEXT((#82385,#82387,#82388))
REPRESENTATION_CONTEXT('','3D')
);
#82385=(
LENGTH_UNIT()
NAMED_UNIT(*)
SI_UNIT(.MILLI.,.METRE.)
);
#82387=(
NAMED_UNIT(*)
PLANE_ANGLE_UNIT()
SI_UNIT($,.RADIAN.)
);
#82388=(
NAMED_UNIT(*)
SI_UNIT($,.STERADIAN.)
SOLID_ANGLE_UNIT()
);
#82393=SHAPE_DEFINITION_REPRESENTATION(#82413,#82469);
#82413=PRODUCT_DEFINITION_SHAPE('',$,#82490);
#82469=SHAPE_REPRESENTATION('',(#31710),#82368);
#82485=PRODUCT_DEFINITION_CONTEXT('part definition',#82547,'design');
#82490=PRODUCT_DEFINITION('2026-10-20-12-38-12-594',
'04_Rotation_Adjuster_Block',#82510,#82485);
#82510=PRODUCT_DEFINITION_FORMATION('',$,#82553);
#82547=APPLICATION_CONTEXT(
'Core Data for Automotive Mechanical Design Process');
#82548=PRODUCT_CONTEXT('part definition',#82547,'mechanical');
#82553=PRODUCT('2026-10-20-12-38-12-594','04_Rotation_Adjuster_Block',$,
(#82548));
#82604=COLOUR_RGB('Dark Blue',0.08,0.2,0.34);
#82605=FILL_AREA_STYLE_COLOUR('',#82604);
#82606=FILL_AREA_STYLE('',(#82605));
#82607=SURFACE_STYLE_FILL_AREA(#82606);
#82608=SURFACE_SIDE_STYLE('',(#82607));
#82609=SURFACE_STYLE_USAGE(.BOTH.,#82608);
#82610=PRESENTATION_STYLE_ASSIGNMENT((#82609));
ENDSEC;
END-ISO-10303-21;
